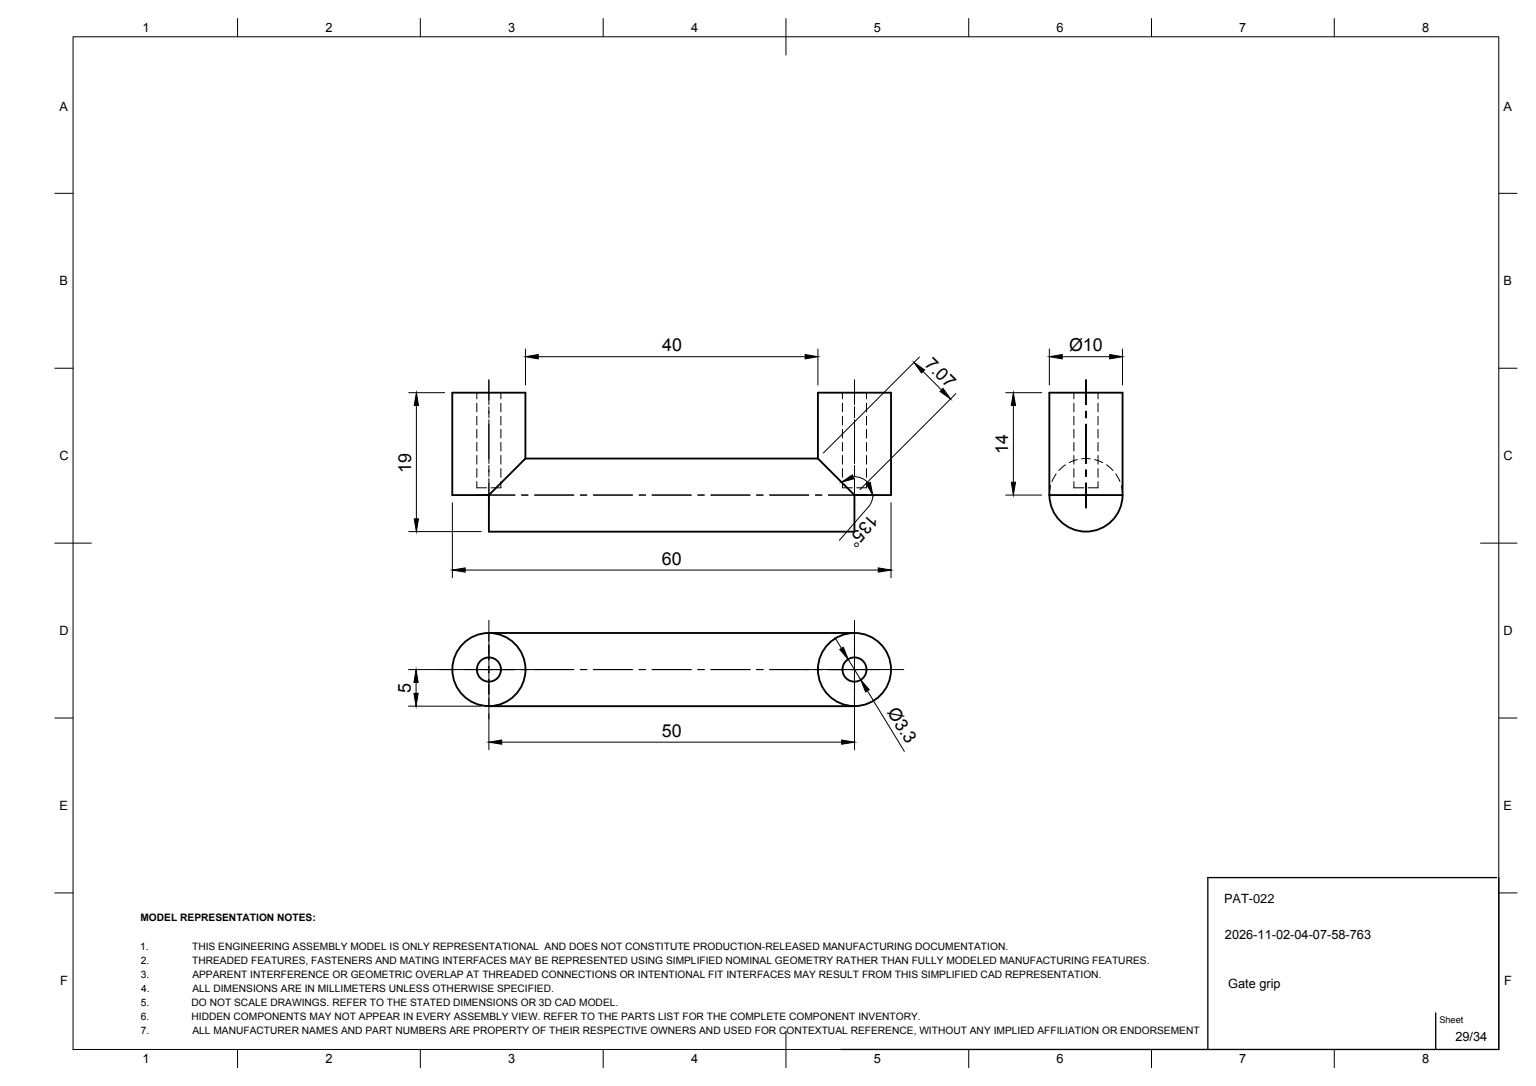
ISO-10303-21;
HEADER;
/* Generated by software containing ST-Developer
 * from STEP Tools, Inc. (www.steptools.com) 
 */

FILE_DESCRIPTION(
/* description */ ('Chute with adjustable gate'),
/* implementation_level */ '2;1');

FILE_NAME(
/* name */ 'Gate grip.step',
/* time_stamp */ '2026-10-27T10:52:28-07:00',
/* author */ (''),
/* organization */ (''),
/* preprocessor_version */ 'ST-DEVELOPER v20.2',
/* originating_system */ 'Autodesk Translation Framework v15.17.0.0',
/* authorisation */ '');

FILE_SCHEMA (('AUTOMOTIVE_DESIGN { 1 0 10303 214 3 1 1 }'));
ENDSEC;

DATA;
#10=MECHANICAL_DESIGN_GEOMETRIC_PRESENTATION_REPRESENTATION('',(#440),#13094);
#325=ELLIPSE('',#8491,0.707106781186548,0.5);
#326=ELLIPSE('',#8501,0.707106781186548,0.5);
#376=SHAPE_REPRESENTATION_RELATIONSHIP('SRR','None',#13278,#408);
#408=ADVANCED_BREP_SHAPE_REPRESENTATION('',(#470),#13087);
#440=STYLED_ITEM('',(#13502),#470);
#470=MANIFOLD_SOLID_BREP('Body1',#7625);
#582=FACE_BOUND('',#1770,.T.);
#583=FACE_BOUND('',#1775,.T.);
#846=PLANE('',#8484);
#847=PLANE('',#8488);
#848=PLANE('',#8493);
#849=PLANE('',#8494);
#850=PLANE('',#8495);
#851=PLANE('',#8502);
#852=PLANE('',#8503);
#853=PLANE('',#8504);
#1241=FACE_OUTER_BOUND('',#1764,.T.);
#1242=FACE_OUTER_BOUND('',#1765,.T.);
#1243=FACE_OUTER_BOUND('',#1766,.T.);
#1244=FACE_OUTER_BOUND('',#1767,.T.);
#1245=FACE_OUTER_BOUND('',#1768,.T.);
#1246=FACE_OUTER_BOUND('',#1769,.T.);
#1247=FACE_OUTER_BOUND('',#1771,.T.);
#1248=FACE_OUTER_BOUND('',#1772,.T.);
#1249=FACE_OUTER_BOUND('',#1773,.T.);
#1250=FACE_OUTER_BOUND('',#1774,.T.);
#1251=FACE_OUTER_BOUND('',#1776,.T.);
#1252=FACE_OUTER_BOUND('',#1777,.T.);
#1253=FACE_OUTER_BOUND('',#1778,.T.);
#1764=EDGE_LOOP('',(#6700,#6701,#6702,#6703));
#1765=EDGE_LOOP('',(#6704));
#1766=EDGE_LOOP('',(#6705,#6706,#6707,#6708));
#1767=EDGE_LOOP('',(#6709));
#1768=EDGE_LOOP('',(#6710,#6711,#6712,#6713,#6714));
#1769=EDGE_LOOP('',(#6715));
#1770=EDGE_LOOP('',(#6716));
#1771=EDGE_LOOP('',(#6717,#6718));
#1772=EDGE_LOOP('',(#6719,#6720,#6721));
#1773=EDGE_LOOP('',(#6722,#6723,#6724,#6725,#6726));
#1774=EDGE_LOOP('',(#6727));
#1775=EDGE_LOOP('',(#6728));
#1776=EDGE_LOOP('',(#6729,#6730));
#1777=EDGE_LOOP('',(#6731,#6732,#6733));
#1778=EDGE_LOOP('',(#6734,#6735,#6736,#6737,#6738,#6739,#6740,#6741));
#2479=LINE('',#12519,#3256);
#2480=LINE('',#12526,#3257);
#2481=LINE('',#12533,#3258);
#2482=LINE('',#12539,#3259);
#2483=LINE('',#12548,#3260);
#2484=LINE('',#12554,#3261);
#2485=LINE('',#12560,#3262);
#3256=VECTOR('',#10311,0.164999999999999);
#3257=VECTOR('',#10320,0.164999999999999);
#3258=VECTOR('',#10329,0.5);
#3259=VECTOR('',#10338,1.);
#3260=VECTOR('',#10349,0.5);
#3261=VECTOR('',#10358,1.);
#3262=VECTOR('',#10367,0.5);
#3550=CIRCLE('',#8482,0.164999999999999);
#3551=CIRCLE('',#8483,0.164999999999999);
#3552=CIRCLE('',#8486,0.164999999999999);
#3553=CIRCLE('',#8487,0.164999999999999);
#3554=CIRCLE('',#8490,0.5);
#3555=CIRCLE('',#8492,0.5);
#3556=CIRCLE('',#8496,0.5);
#3557=CIRCLE('',#8497,0.5);
#3558=CIRCLE('',#8499,0.5);
#3559=CIRCLE('',#8500,0.5);
#3560=CIRCLE('',#8505,0.5);
#3561=CIRCLE('',#8506,0.5);
#4095=VERTEX_POINT('',#12516);
#4096=VERTEX_POINT('',#12518);
#4097=VERTEX_POINT('',#12523);
#4098=VERTEX_POINT('',#12525);
#4099=VERTEX_POINT('',#12530);
#4100=VERTEX_POINT('',#12532);
#4101=VERTEX_POINT('',#12534);
#4102=VERTEX_POINT('',#12541);
#4103=VERTEX_POINT('',#12545);
#4104=VERTEX_POINT('',#12547);
#4105=VERTEX_POINT('',#12549);
#4106=VERTEX_POINT('',#12556);
#4983=EDGE_CURVE('',#4095,#4095,#3550,.T.);
#4984=EDGE_CURVE('',#4095,#4096,#2479,.T.);
#4985=EDGE_CURVE('',#4096,#4096,#3551,.T.);
#4986=EDGE_CURVE('',#4097,#4097,#3552,.T.);
#4987=EDGE_CURVE('',#4097,#4098,#2480,.T.);
#4988=EDGE_CURVE('',#4098,#4098,#3553,.T.);
#4989=EDGE_CURVE('',#4099,#4099,#3554,.T.);
#4990=EDGE_CURVE('',#4099,#4100,#2481,.T.);
#4991=EDGE_CURVE('',#4101,#4100,#325,.T.);
#4992=EDGE_CURVE('',#4101,#4100,#3555,.T.);
#4993=EDGE_CURVE('',#4100,#4101,#2482,.T.);
#4994=EDGE_CURVE('',#4101,#4102,#3556,.T.);
#4995=EDGE_CURVE('',#4102,#4100,#3557,.T.);
#4996=EDGE_CURVE('',#4103,#4103,#3558,.T.);
#4997=EDGE_CURVE('',#4103,#4104,#2483,.T.);
#4998=EDGE_CURVE('',#4104,#4105,#3559,.T.);
#4999=EDGE_CURVE('',#4104,#4105,#326,.T.);
#5000=EDGE_CURVE('',#4105,#4104,#2484,.T.);
#5001=EDGE_CURVE('',#4106,#4104,#3560,.T.);
#5002=EDGE_CURVE('',#4105,#4106,#3561,.T.);
#5003=EDGE_CURVE('',#4102,#4106,#2485,.T.);
#6700=ORIENTED_EDGE('',*,*,#4983,.F.);
#6701=ORIENTED_EDGE('',*,*,#4984,.T.);
#6702=ORIENTED_EDGE('',*,*,#4985,.F.);
#6703=ORIENTED_EDGE('',*,*,#4984,.F.);
#6704=ORIENTED_EDGE('',*,*,#4983,.T.);
#6705=ORIENTED_EDGE('',*,*,#4986,.F.);
#6706=ORIENTED_EDGE('',*,*,#4987,.T.);
#6707=ORIENTED_EDGE('',*,*,#4988,.F.);
#6708=ORIENTED_EDGE('',*,*,#4987,.F.);
#6709=ORIENTED_EDGE('',*,*,#4986,.T.);
#6710=ORIENTED_EDGE('',*,*,#4989,.F.);
#6711=ORIENTED_EDGE('',*,*,#4990,.T.);
#6712=ORIENTED_EDGE('',*,*,#4991,.F.);
#6713=ORIENTED_EDGE('',*,*,#4992,.T.);
#6714=ORIENTED_EDGE('',*,*,#4990,.F.);
#6715=ORIENTED_EDGE('',*,*,#4989,.T.);
#6716=ORIENTED_EDGE('',*,*,#4988,.T.);
#6717=ORIENTED_EDGE('',*,*,#4993,.F.);
#6718=ORIENTED_EDGE('',*,*,#4992,.F.);
#6719=ORIENTED_EDGE('',*,*,#4993,.T.);
#6720=ORIENTED_EDGE('',*,*,#4994,.T.);
#6721=ORIENTED_EDGE('',*,*,#4995,.T.);
#6722=ORIENTED_EDGE('',*,*,#4996,.F.);
#6723=ORIENTED_EDGE('',*,*,#4997,.T.);
#6724=ORIENTED_EDGE('',*,*,#4998,.T.);
#6725=ORIENTED_EDGE('',*,*,#4999,.F.);
#6726=ORIENTED_EDGE('',*,*,#4997,.F.);
#6727=ORIENTED_EDGE('',*,*,#4996,.T.);
#6728=ORIENTED_EDGE('',*,*,#4985,.T.);
#6729=ORIENTED_EDGE('',*,*,#5000,.F.);
#6730=ORIENTED_EDGE('',*,*,#4998,.F.);
#6731=ORIENTED_EDGE('',*,*,#5000,.T.);
#6732=ORIENTED_EDGE('',*,*,#5001,.F.);
#6733=ORIENTED_EDGE('',*,*,#5002,.F.);
#6734=ORIENTED_EDGE('',*,*,#4991,.T.);
#6735=ORIENTED_EDGE('',*,*,#4995,.F.);
#6736=ORIENTED_EDGE('',*,*,#5003,.T.);
#6737=ORIENTED_EDGE('',*,*,#5001,.T.);
#6738=ORIENTED_EDGE('',*,*,#4999,.T.);
#6739=ORIENTED_EDGE('',*,*,#5002,.T.);
#6740=ORIENTED_EDGE('',*,*,#5003,.F.);
#6741=ORIENTED_EDGE('',*,*,#4994,.F.);
#7169=CYLINDRICAL_SURFACE('',#8481,0.164999999999999);
#7170=CYLINDRICAL_SURFACE('',#8485,0.164999999999999);
#7171=CYLINDRICAL_SURFACE('',#8489,0.5);
#7172=CYLINDRICAL_SURFACE('',#8498,0.5);
#7173=CYLINDRICAL_SURFACE('',#8507,0.5);
#7509=ADVANCED_FACE('',(#1241),#7169,.F.);
#7510=ADVANCED_FACE('',(#1242),#846,.T.);
#7511=ADVANCED_FACE('',(#1243),#7170,.F.);
#7512=ADVANCED_FACE('',(#1244),#847,.T.);
#7513=ADVANCED_FACE('',(#1245),#7171,.T.);
#7514=ADVANCED_FACE('',(#1246,#582),#848,.T.);
#7515=ADVANCED_FACE('',(#1247),#849,.F.);
#7516=ADVANCED_FACE('',(#1248),#850,.T.);
#7517=ADVANCED_FACE('',(#1249),#7172,.T.);
#7518=ADVANCED_FACE('',(#1250,#583),#851,.T.);
#7519=ADVANCED_FACE('',(#1251),#852,.F.);
#7520=ADVANCED_FACE('',(#1252),#853,.F.);
#7521=ADVANCED_FACE('',(#1253),#7173,.T.);
#7625=CLOSED_SHELL('',(#7509,#7510,#7511,#7512,#7513,#7514,#7515,#7516,
#7517,#7518,#7519,#7520,#7521));
#8480=AXIS2_PLACEMENT_3D('',#12514,#10305,#10306);
#8481=AXIS2_PLACEMENT_3D('',#12515,#10307,#10308);
#8482=AXIS2_PLACEMENT_3D('',#12517,#10309,#10310);
#8483=AXIS2_PLACEMENT_3D('',#12520,#10312,#10313);
#8484=AXIS2_PLACEMENT_3D('',#12521,#10314,#10315);
#8485=AXIS2_PLACEMENT_3D('',#12522,#10316,#10317);
#8486=AXIS2_PLACEMENT_3D('',#12524,#10318,#10319);
#8487=AXIS2_PLACEMENT_3D('',#12527,#10321,#10322);
#8488=AXIS2_PLACEMENT_3D('',#12528,#10323,#10324);
#8489=AXIS2_PLACEMENT_3D('',#12529,#10325,#10326);
#8490=AXIS2_PLACEMENT_3D('',#12531,#10327,#10328);
#8491=AXIS2_PLACEMENT_3D('',#12535,#10330,#10331);
#8492=AXIS2_PLACEMENT_3D('',#12536,#10332,#10333);
#8493=AXIS2_PLACEMENT_3D('',#12537,#10334,#10335);
#8494=AXIS2_PLACEMENT_3D('',#12538,#10336,#10337);
#8495=AXIS2_PLACEMENT_3D('',#12540,#10339,#10340);
#8496=AXIS2_PLACEMENT_3D('',#12542,#10341,#10342);
#8497=AXIS2_PLACEMENT_3D('',#12543,#10343,#10344);
#8498=AXIS2_PLACEMENT_3D('',#12544,#10345,#10346);
#8499=AXIS2_PLACEMENT_3D('',#12546,#10347,#10348);
#8500=AXIS2_PLACEMENT_3D('',#12550,#10350,#10351);
#8501=AXIS2_PLACEMENT_3D('',#12551,#10352,#10353);
#8502=AXIS2_PLACEMENT_3D('',#12552,#10354,#10355);
#8503=AXIS2_PLACEMENT_3D('',#12553,#10356,#10357);
#8504=AXIS2_PLACEMENT_3D('',#12555,#10359,#10360);
#8505=AXIS2_PLACEMENT_3D('',#12557,#10361,#10362);
#8506=AXIS2_PLACEMENT_3D('',#12558,#10363,#10364);
#8507=AXIS2_PLACEMENT_3D('',#12559,#10365,#10366);
#10305=DIRECTION('axis',(0.,0.,1.));
#10306=DIRECTION('refdir',(1.,0.,0.));
#10307=DIRECTION('center_axis',(1.,0.,0.));
#10308=DIRECTION('ref_axis',(0.,0.,-1.));
#10309=DIRECTION('center_axis',(1.,0.,0.));
#10310=DIRECTION('ref_axis',(0.,0.,-1.));
#10311=DIRECTION('',(1.,0.,0.));
#10312=DIRECTION('center_axis',(-1.,0.,0.));
#10313=DIRECTION('ref_axis',(0.,0.,-1.));
#10314=DIRECTION('center_axis',(1.,0.,0.));
#10315=DIRECTION('ref_axis',(0.,0.,-1.));
#10316=DIRECTION('center_axis',(1.,0.,0.));
#10317=DIRECTION('ref_axis',(0.,0.,-1.));
#10318=DIRECTION('center_axis',(1.,0.,0.));
#10319=DIRECTION('ref_axis',(0.,0.,-1.));
#10320=DIRECTION('',(1.,0.,0.));
#10321=DIRECTION('center_axis',(-1.,0.,0.));
#10322=DIRECTION('ref_axis',(0.,0.,-1.));
#10323=DIRECTION('center_axis',(1.,0.,0.));
#10324=DIRECTION('ref_axis',(0.,0.,-1.));
#10325=DIRECTION('center_axis',(1.,0.,0.));
#10326=DIRECTION('ref_axis',(0.,0.,-1.));
#10327=DIRECTION('center_axis',(1.,0.,0.));
#10328=DIRECTION('ref_axis',(0.,0.,-1.));
#10329=DIRECTION('',(-1.,0.,0.));
#10330=DIRECTION('center_axis',(-0.707106781186548,-0.707106781186548,0.));
#10331=DIRECTION('ref_axis',(-0.707106781186547,0.707106781186547,0.));
#10332=DIRECTION('center_axis',(1.,0.,0.));
#10333=DIRECTION('ref_axis',(0.,0.,-1.));
#10334=DIRECTION('center_axis',(1.,0.,0.));
#10335=DIRECTION('ref_axis',(0.,0.,-1.));
#10336=DIRECTION('center_axis',(1.,0.,0.));
#10337=DIRECTION('ref_axis',(0.,0.,-1.));
#10338=DIRECTION('',(0.,0.,-1.));
#10339=DIRECTION('center_axis',(0.,1.,0.));
#10340=DIRECTION('ref_axis',(1.,0.,0.));
#10341=DIRECTION('center_axis',(0.,1.,0.));
#10342=DIRECTION('ref_axis',(1.,0.,0.));
#10343=DIRECTION('center_axis',(0.,1.,0.));
#10344=DIRECTION('ref_axis',(1.,0.,0.));
#10345=DIRECTION('center_axis',(1.,0.,0.));
#10346=DIRECTION('ref_axis',(0.,0.,-1.));
#10347=DIRECTION('center_axis',(1.,0.,0.));
#10348=DIRECTION('ref_axis',(0.,0.,-1.));
#10349=DIRECTION('',(-1.,0.,0.));
#10350=DIRECTION('center_axis',(1.,0.,0.));
#10351=DIRECTION('ref_axis',(0.,0.,-1.));
#10352=DIRECTION('center_axis',(-0.707106781186548,0.707106781186548,0.));
#10353=DIRECTION('ref_axis',(0.707106781186547,0.707106781186547,0.));
#10354=DIRECTION('center_axis',(1.,0.,0.));
#10355=DIRECTION('ref_axis',(0.,0.,-1.));
#10356=DIRECTION('center_axis',(1.,0.,0.));
#10357=DIRECTION('ref_axis',(0.,0.,-1.));
#10358=DIRECTION('',(0.,0.,1.));
#10359=DIRECTION('center_axis',(0.,1.,0.));
#10360=DIRECTION('ref_axis',(1.,0.,0.));
#10361=DIRECTION('center_axis',(0.,1.,0.));
#10362=DIRECTION('ref_axis',(1.,0.,0.));
#10363=DIRECTION('center_axis',(0.,1.,0.));
#10364=DIRECTION('ref_axis',(1.,0.,0.));
#10365=DIRECTION('center_axis',(0.,1.,0.));
#10366=DIRECTION('ref_axis',(1.,0.,0.));
#10367=DIRECTION('',(0.,-1.,0.));
#12514=CARTESIAN_POINT('',(0.,0.,0.));
#12515=CARTESIAN_POINT('Origin',(-2.9,-2.5,15.));
#12516=CARTESIAN_POINT('',(-2.9,-2.5,15.165));
#12517=CARTESIAN_POINT('Origin',(-2.9,-2.5,15.));
#12518=CARTESIAN_POINT('',(-1.6,-2.5,15.165));
#12519=CARTESIAN_POINT('',(-2.9,-2.5,15.165));
#12520=CARTESIAN_POINT('Origin',(-1.6,-2.5,15.));
#12521=CARTESIAN_POINT('Origin',(-2.9,-2.5,15.));
#12522=CARTESIAN_POINT('Origin',(-2.9,2.5,15.));
#12523=CARTESIAN_POINT('',(-2.9,2.5,15.165));
#12524=CARTESIAN_POINT('Origin',(-2.9,2.5,15.));
#12525=CARTESIAN_POINT('',(-1.6,2.5,15.165));
#12526=CARTESIAN_POINT('',(-2.9,2.5,15.165));
#12527=CARTESIAN_POINT('Origin',(-1.6,2.5,15.));
#12528=CARTESIAN_POINT('Origin',(-2.9,2.5,15.));
#12529=CARTESIAN_POINT('Origin',(-3.,2.5,15.));
#12530=CARTESIAN_POINT('',(-1.6,2.5,15.5));
#12531=CARTESIAN_POINT('Origin',(-1.6,2.5,15.));
#12532=CARTESIAN_POINT('',(-3.,2.5,15.5));
#12533=CARTESIAN_POINT('',(-3.,2.5,15.5));
#12534=CARTESIAN_POINT('',(-3.,2.5,14.5));
#12535=CARTESIAN_POINT('Origin',(-3.,2.5,15.));
#12536=CARTESIAN_POINT('Origin',(-3.,2.5,15.));
#12537=CARTESIAN_POINT('Origin',(-1.6,2.5,15.));
#12538=CARTESIAN_POINT('Origin',(-3.,2.5,15.));
#12539=CARTESIAN_POINT('',(-3.,2.5,15.));
#12540=CARTESIAN_POINT('Origin',(-3.,2.5,15.));
#12541=CARTESIAN_POINT('',(-3.5,2.5,15.));
#12542=CARTESIAN_POINT('Origin',(-3.,2.5,15.));
#12543=CARTESIAN_POINT('Origin',(-3.,2.5,15.));
#12544=CARTESIAN_POINT('Origin',(-3.,-2.5,15.));
#12545=CARTESIAN_POINT('',(-1.6,-2.5,15.5));
#12546=CARTESIAN_POINT('Origin',(-1.6,-2.5,15.));
#12547=CARTESIAN_POINT('',(-3.,-2.5,15.5));
#12548=CARTESIAN_POINT('',(-3.,-2.5,15.5));
#12549=CARTESIAN_POINT('',(-3.,-2.5,14.5));
#12550=CARTESIAN_POINT('Origin',(-3.,-2.5,15.));
#12551=CARTESIAN_POINT('Origin',(-3.,-2.5,15.));
#12552=CARTESIAN_POINT('Origin',(-1.6,-2.5,15.));
#12553=CARTESIAN_POINT('Origin',(-3.,-2.5,15.));
#12554=CARTESIAN_POINT('',(-3.,-2.5,15.));
#12555=CARTESIAN_POINT('Origin',(-3.,-2.5,15.));
#12556=CARTESIAN_POINT('',(-3.5,-2.5,15.));
#12557=CARTESIAN_POINT('Origin',(-3.,-2.5,15.));
#12558=CARTESIAN_POINT('Origin',(-3.,-2.5,15.));
#12559=CARTESIAN_POINT('Origin',(-3.,-2.5,15.));
#12560=CARTESIAN_POINT('',(-3.5,-2.5,15.));
#13050=UNCERTAINTY_MEASURE_WITH_UNIT(LENGTH_MEASURE(0.001),#13095,
'DISTANCE_ACCURACY_VALUE',
'Maximum model space distance between geometric entities at asserted c
onnectivities');
#13057=UNCERTAINTY_MEASURE_WITH_UNIT(LENGTH_MEASURE(0.001),#13095,
'DISTANCE_ACCURACY_VALUE',
'Maximum model space distance between geometric entities at asserted c
onnectivities');
#13087=(
GEOMETRIC_REPRESENTATION_CONTEXT(3)
GLOBAL_UNCERTAINTY_ASSIGNED_CONTEXT((#13050))
GLOBAL_UNIT_ASSIGNED_CONTEXT((#13095,#13097,#13098))
REPRESENTATION_CONTEXT('','3D')
);
#13094=(
GEOMETRIC_REPRESENTATION_CONTEXT(3)
GLOBAL_UNCERTAINTY_ASSIGNED_CONTEXT((#13057))
GLOBAL_UNIT_ASSIGNED_CONTEXT((#13095,#13097,#13098))
REPRESENTATION_CONTEXT('','3D')
);
#13095=(
LENGTH_UNIT()
NAMED_UNIT(*)
SI_UNIT(.CENTI.,.METRE.)
);
#13097=(
NAMED_UNIT(*)
PLANE_ANGLE_UNIT()
SI_UNIT($,.RADIAN.)
);
#13098=(
NAMED_UNIT(*)
SI_UNIT($,.STERADIAN.)
SOLID_ANGLE_UNIT()
);
#13128=SHAPE_DEFINITION_REPRESENTATION(#13164,#13278);
#13164=PRODUCT_DEFINITION_SHAPE('',$,#13315);
#13278=SHAPE_REPRESENTATION('',(#8480),#13087);
#13285=PRODUCT_DEFINITION_CONTEXT('part definition',#13395,'design');
#13315=PRODUCT_DEFINITION('Gate grip','Gate grip',#13351,#13285);
#13351=PRODUCT_DEFINITION_FORMATION('',$,#13426);
#13395=APPLICATION_CONTEXT(
'Core Data for Automotive Mechanical Design Process');
#13396=PRODUCT_CONTEXT('part definition',#13395,'mechanical');
#13426=PRODUCT('Gate grip','Gate grip','Gate grip',(#13396));
#13496=COLOUR_RGB('Black',0.12,0.14,0.17);
#13497=FILL_AREA_STYLE_COLOUR('',#13496);
#13498=FILL_AREA_STYLE('',(#13497));
#13499=SURFACE_STYLE_FILL_AREA(#13498);
#13500=SURFACE_SIDE_STYLE('',(#13499));
#13501=SURFACE_STYLE_USAGE(.BOTH.,#13500);
#13502=PRESENTATION_STYLE_ASSIGNMENT((#13501));
ENDSEC;
END-ISO-10303-21;
